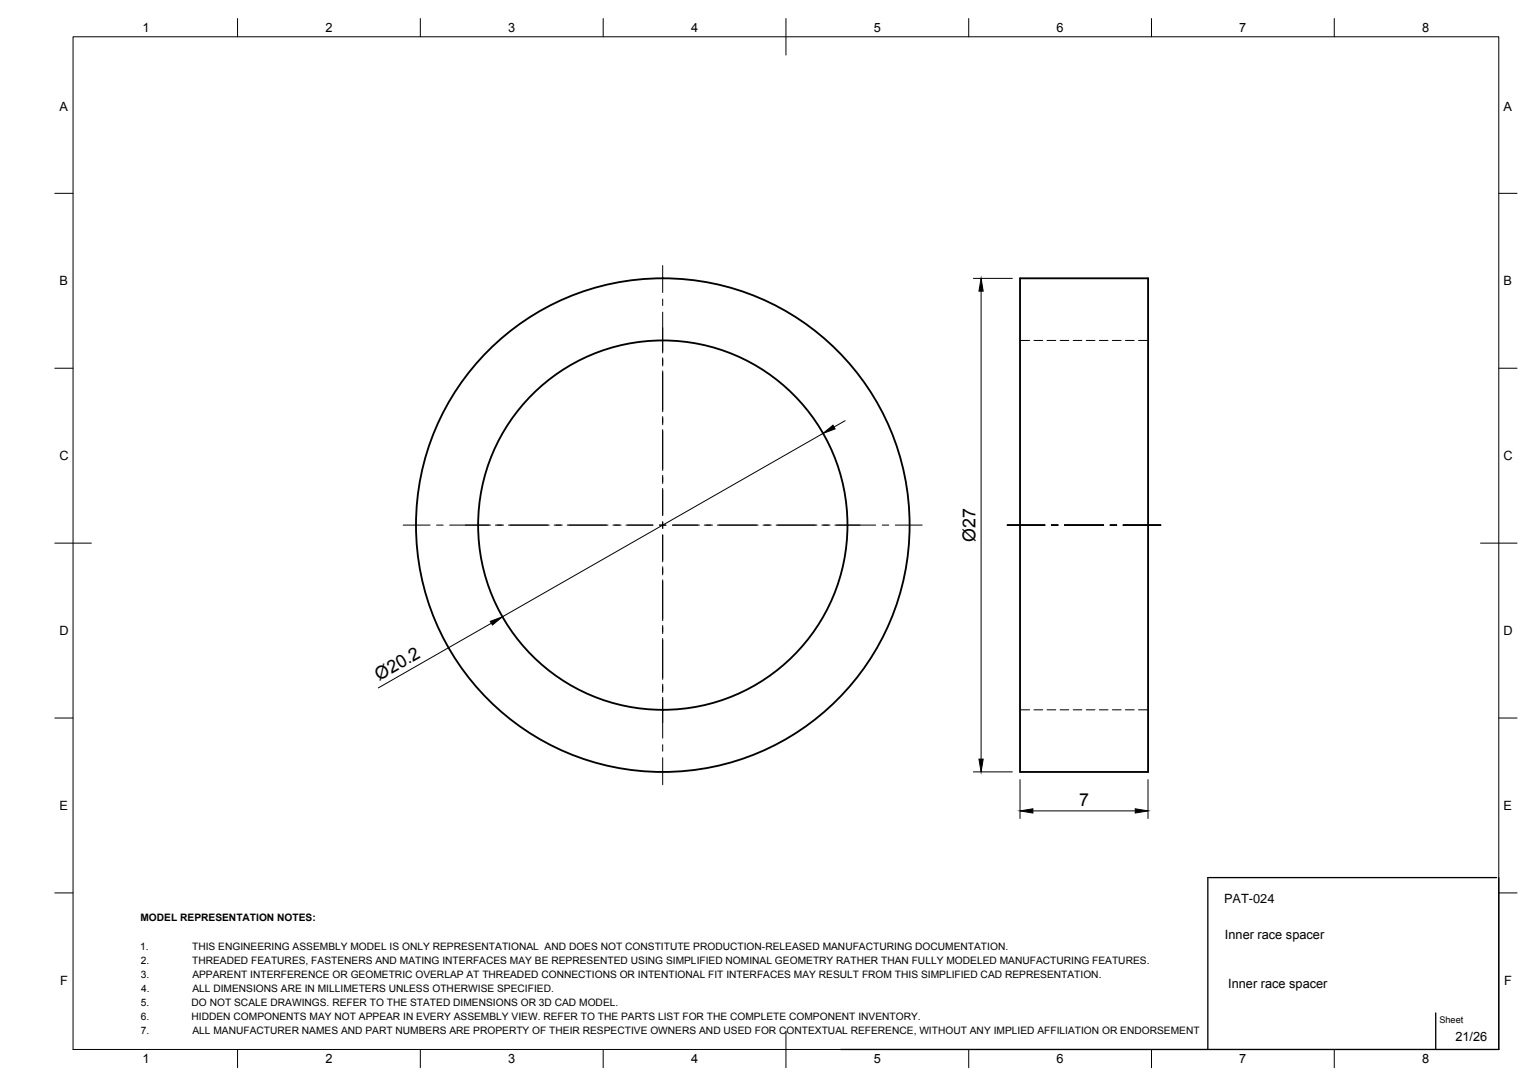
ISO-10303-21;
HEADER;
/* Generated by software containing ST-Developer
 * from STEP Tools, Inc. (www.steptools.com) 
 */

FILE_DESCRIPTION(
/* description */ ('Compact handwheel screw vise'),
/* implementation_level */ '2;1');

FILE_NAME(
/* name */ 'Inner race spacer.step',
/* time_stamp */ '2026-10-29T16:08:22-07:00',
/* author */ (''),
/* organization */ (''),
/* preprocessor_version */ 'ST-DEVELOPER v20.2',
/* originating_system */ 'Autodesk Translation Framework v15.17.0.0',
/* authorisation */ '');

FILE_SCHEMA (('AUTOMOTIVE_DESIGN { 1 0 10303 214 3 1 1 }'));
ENDSEC;

DATA;
#10=MECHANICAL_DESIGN_GEOMETRIC_PRESENTATION_REPRESENTATION('',(#671),#25074);
#607=SHAPE_REPRESENTATION_RELATIONSHIP('SRR','None',#25218,#635);
#635=ADVANCED_BREP_SHAPE_REPRESENTATION('',(#704),#25065);
#671=STYLED_ITEM('',(#25439),#704);
#704=MANIFOLD_SOLID_BREP('Body1',#8082);
#802=FACE_BOUND('',#1970,.T.);
#803=FACE_BOUND('',#1972,.T.);
#962=PLANE('',#9050);
#963=PLANE('',#9051);
#1407=FACE_OUTER_BOUND('',#1967,.T.);
#1408=FACE_OUTER_BOUND('',#1968,.T.);
#1409=FACE_OUTER_BOUND('',#1969,.T.);
#1410=FACE_OUTER_BOUND('',#1971,.T.);
#1967=EDGE_LOOP('',(#7035,#7036,#7037,#7038));
#1968=EDGE_LOOP('',(#7039,#7040,#7041,#7042));
#1969=EDGE_LOOP('',(#7043));
#1970=EDGE_LOOP('',(#7044));
#1971=EDGE_LOOP('',(#7045));
#1972=EDGE_LOOP('',(#7046));
#2469=LINE('',#24524,#2977);
#2470=LINE('',#24530,#2978);
#2977=VECTOR('',#10901,1.01);
#2978=VECTOR('',#10908,1.35);
#3289=CIRCLE('',#9045,1.01);
#3290=CIRCLE('',#9046,1.01);
#3291=CIRCLE('',#9048,1.35);
#3292=CIRCLE('',#9049,1.35);
#3964=VERTEX_POINT('',#24521);
#3965=VERTEX_POINT('',#24523);
#3966=VERTEX_POINT('',#24527);
#3967=VERTEX_POINT('',#24529);
#5004=EDGE_CURVE('',#3964,#3964,#3289,.T.);
#5005=EDGE_CURVE('',#3964,#3965,#2469,.T.);
#5006=EDGE_CURVE('',#3965,#3965,#3290,.T.);
#5007=EDGE_CURVE('',#3966,#3966,#3291,.T.);
#5008=EDGE_CURVE('',#3966,#3967,#2470,.T.);
#5009=EDGE_CURVE('',#3967,#3967,#3292,.T.);
#7035=ORIENTED_EDGE('',*,*,#5004,.F.);
#7036=ORIENTED_EDGE('',*,*,#5005,.T.);
#7037=ORIENTED_EDGE('',*,*,#5006,.T.);
#7038=ORIENTED_EDGE('',*,*,#5005,.F.);
#7039=ORIENTED_EDGE('',*,*,#5007,.F.);
#7040=ORIENTED_EDGE('',*,*,#5008,.T.);
#7041=ORIENTED_EDGE('',*,*,#5009,.T.);
#7042=ORIENTED_EDGE('',*,*,#5008,.F.);
#7043=ORIENTED_EDGE('',*,*,#5007,.T.);
#7044=ORIENTED_EDGE('',*,*,#5004,.T.);
#7045=ORIENTED_EDGE('',*,*,#5009,.F.);
#7046=ORIENTED_EDGE('',*,*,#5006,.F.);
#7563=CYLINDRICAL_SURFACE('',#9044,1.01);
#7564=CYLINDRICAL_SURFACE('',#9047,1.35);
#7977=ADVANCED_FACE('',(#1407),#7563,.F.);
#7978=ADVANCED_FACE('',(#1408),#7564,.T.);
#7979=ADVANCED_FACE('',(#1409,#802),#962,.T.);
#7980=ADVANCED_FACE('',(#1410,#803),#963,.F.);
#8082=CLOSED_SHELL('',(#7977,#7978,#7979,#7980));
#9043=AXIS2_PLACEMENT_3D('',#24519,#10895,#10896);
#9044=AXIS2_PLACEMENT_3D('',#24520,#10897,#10898);
#9045=AXIS2_PLACEMENT_3D('',#24522,#10899,#10900);
#9046=AXIS2_PLACEMENT_3D('',#24525,#10902,#10903);
#9047=AXIS2_PLACEMENT_3D('',#24526,#10904,#10905);
#9048=AXIS2_PLACEMENT_3D('',#24528,#10906,#10907);
#9049=AXIS2_PLACEMENT_3D('',#24531,#10909,#10910);
#9050=AXIS2_PLACEMENT_3D('',#24532,#10911,#10912);
#9051=AXIS2_PLACEMENT_3D('',#24533,#10913,#10914);
#10895=DIRECTION('axis',(0.,0.,1.));
#10896=DIRECTION('refdir',(1.,0.,0.));
#10897=DIRECTION('center_axis',(1.,0.,0.));
#10898=DIRECTION('ref_axis',(0.,0.,-1.));
#10899=DIRECTION('center_axis',(-1.,0.,0.));
#10900=DIRECTION('ref_axis',(0.,0.,-1.));
#10901=DIRECTION('',(-1.,0.,0.));
#10902=DIRECTION('center_axis',(-1.,0.,0.));
#10903=DIRECTION('ref_axis',(0.,0.,-1.));
#10904=DIRECTION('center_axis',(1.,0.,0.));
#10905=DIRECTION('ref_axis',(0.,0.,-1.));
#10906=DIRECTION('center_axis',(1.,0.,0.));
#10907=DIRECTION('ref_axis',(0.,0.,-1.));
#10908=DIRECTION('',(-1.,0.,0.));
#10909=DIRECTION('center_axis',(1.,0.,0.));
#10910=DIRECTION('ref_axis',(0.,0.,-1.));
#10911=DIRECTION('center_axis',(1.,0.,0.));
#10912=DIRECTION('ref_axis',(0.,0.,-1.));
#10913=DIRECTION('center_axis',(1.,0.,0.));
#10914=DIRECTION('ref_axis',(0.,0.,-1.));
#24519=CARTESIAN_POINT('',(0.,0.,0.));
#24520=CARTESIAN_POINT('Origin',(24.7,0.,4.));
#24521=CARTESIAN_POINT('',(25.4,-1.23689326713883E-16,5.01));
#24522=CARTESIAN_POINT('Origin',(25.4,0.,4.));
#24523=CARTESIAN_POINT('',(24.7,-1.23689326713883E-16,5.01));
#24524=CARTESIAN_POINT('',(24.7,-1.23689326713883E-16,5.01));
#24525=CARTESIAN_POINT('Origin',(24.7,0.,4.));
#24526=CARTESIAN_POINT('Origin',(24.7,0.,4.));
#24527=CARTESIAN_POINT('',(25.4,-1.65327317884893E-16,5.35));
#24528=CARTESIAN_POINT('Origin',(25.4,0.,4.));
#24529=CARTESIAN_POINT('',(24.7,-1.65327317884893E-16,5.35));
#24530=CARTESIAN_POINT('',(24.7,-1.65327317884893E-16,5.35));
#24531=CARTESIAN_POINT('Origin',(24.7,0.,4.));
#24532=CARTESIAN_POINT('Origin',(25.4,0.,4.));
#24533=CARTESIAN_POINT('Origin',(24.7,0.,4.));
#25031=UNCERTAINTY_MEASURE_WITH_UNIT(LENGTH_MEASURE(0.001),#25075,
'DISTANCE_ACCURACY_VALUE',
'Maximum model space distance between geometric entities at asserted c
onnectivities');
#25040=UNCERTAINTY_MEASURE_WITH_UNIT(LENGTH_MEASURE(0.001),#25075,
'DISTANCE_ACCURACY_VALUE',
'Maximum model space distance between geometric entities at asserted c
onnectivities');
#25065=(
GEOMETRIC_REPRESENTATION_CONTEXT(3)
GLOBAL_UNCERTAINTY_ASSIGNED_CONTEXT((#25031))
GLOBAL_UNIT_ASSIGNED_CONTEXT((#25075,#25077,#25078))
REPRESENTATION_CONTEXT('','3D')
);
#25074=(
GEOMETRIC_REPRESENTATION_CONTEXT(3)
GLOBAL_UNCERTAINTY_ASSIGNED_CONTEXT((#25040))
GLOBAL_UNIT_ASSIGNED_CONTEXT((#25075,#25077,#25078))
REPRESENTATION_CONTEXT('','3D')
);
#25075=(
LENGTH_UNIT()
NAMED_UNIT(*)
SI_UNIT(.CENTI.,.METRE.)
);
#25077=(
NAMED_UNIT(*)
PLANE_ANGLE_UNIT()
SI_UNIT($,.RADIAN.)
);
#25078=(
NAMED_UNIT(*)
SI_UNIT($,.STERADIAN.)
SOLID_ANGLE_UNIT()
);
#25103=SHAPE_DEFINITION_REPRESENTATION(#25152,#25218);
#25152=PRODUCT_DEFINITION_SHAPE('',$,#25252);
#25218=SHAPE_REPRESENTATION('',(#9043),#25065);
#25227=PRODUCT_DEFINITION_CONTEXT('part definition',#25328,'design');
#25252=PRODUCT_DEFINITION('Inner race spacer','Inner race spacer',#25285,
#25227);
#25285=PRODUCT_DEFINITION_FORMATION('',$,#25354);
#25328=APPLICATION_CONTEXT(
'Core Data for Automotive Mechanical Design Process');
#25329=PRODUCT_CONTEXT('part definition',#25328,'mechanical');
#25354=PRODUCT('Inner race spacer','Inner race spacer',
'Inner race spacer',(#25329));
#25433=COLOUR_RGB('Grey',0.48,0.52,0.57);
#25434=FILL_AREA_STYLE_COLOUR('',#25433);
#25435=FILL_AREA_STYLE('',(#25434));
#25436=SURFACE_STYLE_FILL_AREA(#25435);
#25437=SURFACE_SIDE_STYLE('',(#25436));
#25438=SURFACE_STYLE_USAGE(.BOTH.,#25437);
#25439=PRESENTATION_STYLE_ASSIGNMENT((#25438));
ENDSEC;
END-ISO-10303-21;
